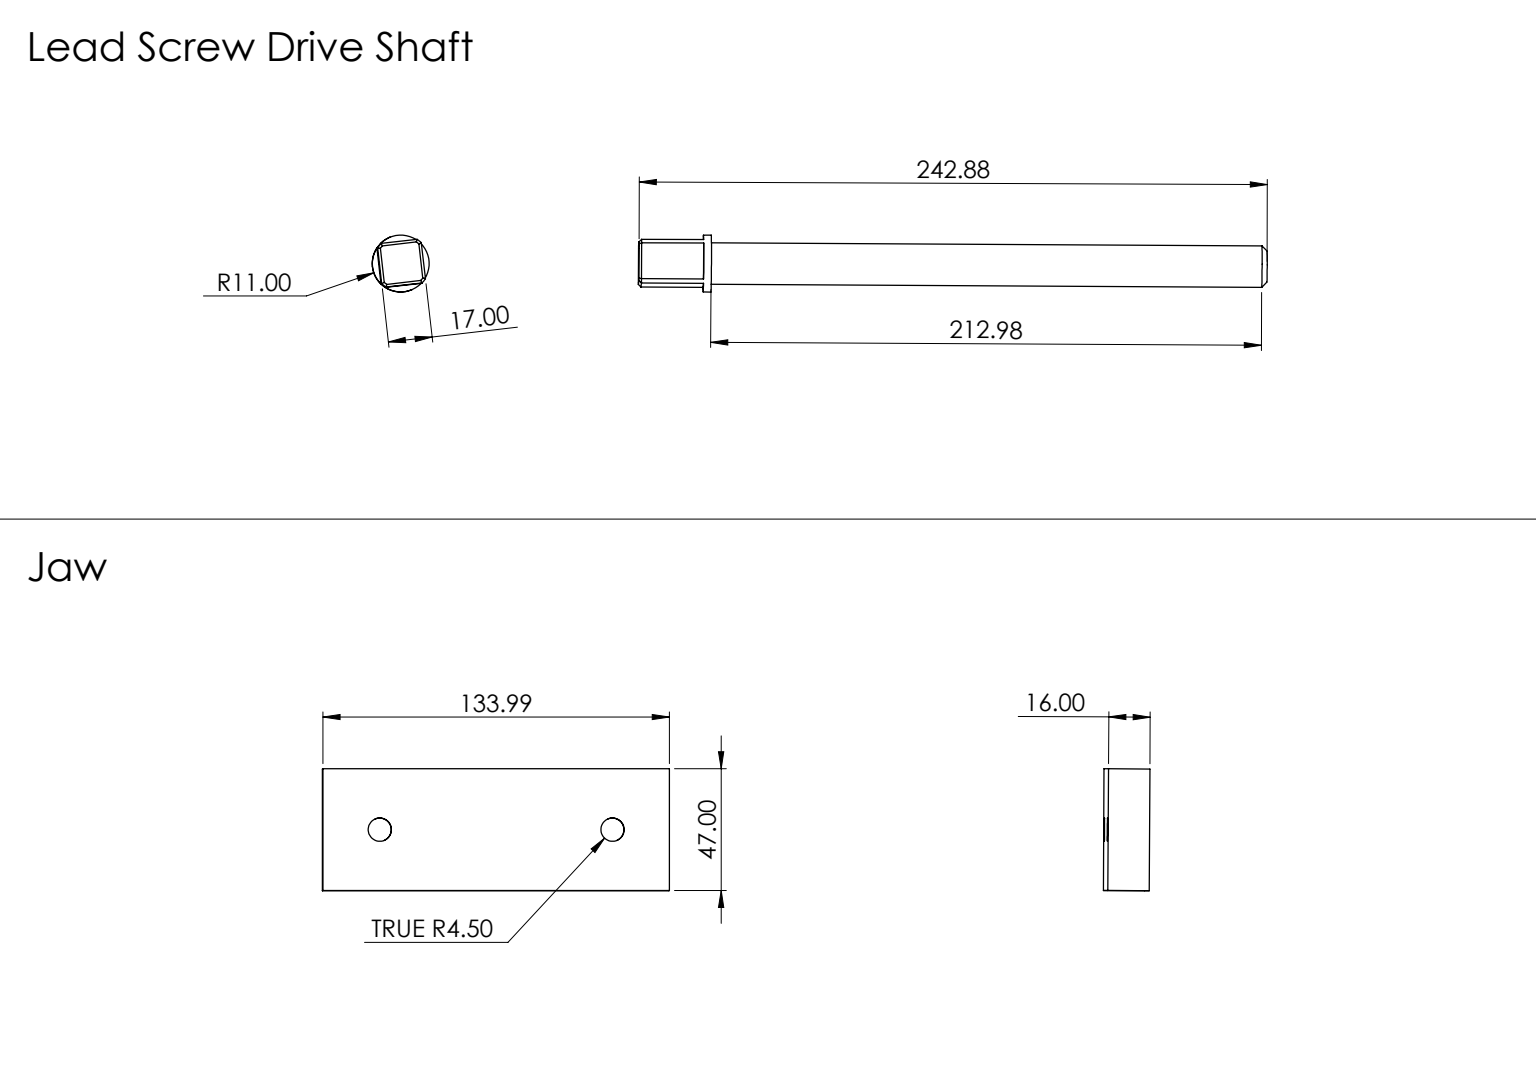
ISO-10303-21;
HEADER;
FILE_DESCRIPTION (('STEP AP214'),
    '1' );
FILE_NAME ('Jaw.step',
    '2026-10-09T10:51:02',
    ( '' ),
    ( '' ),
    'SwSTEP 2.0',
    'SolidWorks 2026',
    '' );
FILE_SCHEMA (( 'AUTOMOTIVE_DESIGN' ));
ENDSEC;

DATA;
#34=DIRECTION ( 'NONE',  ( -7.125109674081160920E-05, 0.9999848031710253382, -0.005512562950849312846 ) ) ;
#150=DIRECTION ( 'NONE',  ( -7.125109674118361251E-05, 0.9999848031710253382, -0.005512562950849477644 ) ) ;
#162=FACE_BOUND ( 'NONE', #20297, .T. ) ;
#274=ORIENTED_EDGE ( 'NONE', *, *, #11916, .F. ) ;
#303=VECTOR ( 'NONE', #7071, 999.9999999999998863 ) ;
#315=CARTESIAN_POINT ( 'NONE',  ( 67.23655452815148692, 145.1029152106949027, 17.86880078497820179 ) ) ;
#352=EDGE_LOOP ( 'NONE', ( #16374, #6015 ) ) ;
#357=ORIENTED_EDGE ( 'NONE', *, *, #20567, .F. ) ;
#370=AXIS2_PLACEMENT_3D ( 'NONE', #9762, #6313, #11942 ) ;
#420=DIRECTION ( 'NONE',  ( -7.125109674025824596E-05, 0.9999848031710253382, -0.005512562950848693549 ) ) ;
#429=LINE ( 'NONE', #2033, #16330 ) ;
#449=AXIS2_PLACEMENT_3D ( 'NONE', #14945, #15170, #16666 ) ;
#652=ORIENTED_EDGE ( 'NONE', *, *, #21301, .F. ) ;
#687=LINE ( 'NONE', #9519, #12271 ) ;
#716=DIRECTION ( 'NONE',  ( -7.125109674025824596E-05, 0.9999848031710253382, -0.005512562950848693549 ) ) ;
#813=UNCERTAINTY_MEASURE_WITH_UNIT (LENGTH_MEASURE( 1.000000000000000082E-05 ), #17647, 'distance_accuracy_value', 'NONE');
#839=VECTOR ( 'NONE', #4920, 999.9999999999998863 ) ;
#857=ORIENTED_EDGE ( 'NONE', *, *, #10212, .F. ) ;
#859=AXIS2_PLACEMENT_3D ( 'NONE', #22163, #3207, #9893 ) ;
#896=DIRECTION ( 'NONE',  ( -7.125109674081160920E-05, 0.9999848031710253382, -0.005512562950849312846 ) ) ;
#960=ADVANCED_FACE ( 'NONE', ( #15043 ), #20731, .F. ) ;
#993=ORIENTED_EDGE ( 'NONE', *, *, #20376, .T. ) ;
#1015=ORIENTED_EDGE ( 'NONE', *, *, #13140, .F. ) ;
#1210=EDGE_CURVE ( 'NONE', #16785, #22481, #5763, .T. ) ;
#1305=CARTESIAN_POINT ( 'NONE',  ( -44.65183966190961939, 161.1467762486291520, 27.22731394492822687 ) ) ;
#1395=DIRECTION ( 'NONE',  ( 1.000000000000000000, 0.000000000000000000, 0.000000000000000000 ) ) ;
#1432=EDGE_LOOP ( 'NONE', ( #10019, #11509, #17070, #14854 ) ) ;
#1475=CARTESIAN_POINT ( 'NONE',  ( 49.83973329503886873, 168.6466622724117599, 25.96463831280822632 ) ) ;
#1540=( GEOMETRIC_REPRESENTATION_CONTEXT ( 3 ) GLOBAL_UNCERTAINTY_ASSIGNED_CONTEXT ( ( #813 ) ) GLOBAL_UNIT_ASSIGNED_CONTEXT ( ( #17647, #10405, #3847 ) ) REPRESENTATION_CONTEXT ( 'NONE', 'WORKASPACE' ) );
#1577=CARTESIAN_POINT ( 'NONE',  ( 45.44318007003697346, 173.1906980738791617, 33.99720069194405170 ) ) ;
#1592=AXIS2_PLACEMENT_3D ( 'NONE', #10762, #9016, #16064 ) ;
#1663=ORIENTED_EDGE ( 'NONE', *, *, #8994, .T. ) ;
#1682=SHAPE_REPRESENTATION_RELATIONSHIP ( 'NONE' , 'NONE' ,  #3137, #19759 ) ;
#1704=LINE ( 'NONE', #11119, #17313 ) ;
#1846=DIRECTION ( 'NONE',  ( -0.01292394549866741384, -0.005513023399720269613, -0.9999012842304692006 ) ) ;
#1876=EDGE_CURVE ( 'NONE', #11555, #17908, #8775, .T. ) ;
#1910=EDGE_CURVE ( 'NONE', #1979, #4369, #21194, .T. ) ;
#1979=VERTEX_POINT ( 'NONE', #8220 ) ;
#1998=PLANE ( 'NONE',  #3714 ) ;
#2033=CARTESIAN_POINT ( 'NONE',  ( 45.23703820192896075, 164.1026264709443865, 18.04839321081418291 ) ) ;
#2042=DIRECTION ( 'NONE',  ( -0.01292394549866741384, -0.005513023399720269613, -0.9999012842304692006 ) ) ;
#2146=CARTESIAN_POINT ( 'NONE',  ( 45.23671757199362986, 168.6025580852140138, 18.02358667753535926 ) ) ;
#2182=ORIENTED_EDGE ( 'NONE', *, *, #8536, .T. ) ;
#2189=CARTESIAN_POINT ( 'NONE',  ( 45.34010913598296355, 168.6466622724117599, 26.02279695137911020 ) ) ;
#2195=CARTESIAN_POINT ( 'NONE',  ( -44.54930311108117280, 173.1906980738792186, 35.16037346336178615 ) ) ;
#2208=ORIENTED_EDGE ( 'NONE', *, *, #19527, .F. ) ;
#2265=AXIS2_PLACEMENT_3D ( 'NONE', #6781, #4820, #15212 ) ;
#2299=AXIS2_PLACEMENT_3D ( 'NONE', #18895, #10594, #12683 ) ;
#2309=VERTEX_POINT ( 'NONE', #20349 ) ;
#2386=CARTESIAN_POINT ( 'NONE',  ( 0.4472591094132349898, 168.6907664596095628, 34.60359361093173902 ) ) ;
#2477=CARTESIAN_POINT ( 'NONE',  ( -66.75225376373553843, 145.1029152106950164, 19.60063580020017326 ) ) ;
#2488=DIRECTION ( 'NONE',  ( -0.01292394549866741384, -0.005513023399720270480, -0.9999012842304693116 ) ) ;
#2502=DIRECTION ( 'NONE',  ( 0.01292394549866741557, 0.005513023399720270480, 0.9999012842304693116 ) ) ;
#2503=EDGE_CURVE ( 'NONE', #1979, #11555, #13540, .T. ) ;
#2515=DIRECTION ( 'NONE',  ( -7.125109674025824596E-05, 0.9999848031710253382, -0.005512562950849464634 ) ) ;
#2611=ADVANCED_FACE ( 'NONE', ( #19733 ), #11028, .F. ) ;
#2640=DIRECTION ( 'NONE',  ( -7.125109674118361251E-05, 0.9999848031710253382, -0.005512562950849477644 ) ) ;
#2688=EDGE_CURVE ( 'NONE', #17908, #4369, #17967, .T. ) ;
#2724=FACE_OUTER_BOUND ( 'NONE', #16793, .T. ) ;
#2742=EDGE_LOOP ( 'NONE', ( #5687, #11839, #12737, #13981 ) ) ;
#2858=DIRECTION ( 'NONE',  ( -0.01292394549866741384, -0.005513023399720269613, -0.9999012842304692006 ) ) ;
#2946=CARTESIAN_POINT ( 'NONE',  ( -44.75576560912451640, 168.6025580852140706, 19.18675944895310082 ) ) ;
#2950=AXIS2_PLACEMENT_3D ( 'NONE', #15940, #17886, #10862 ) ;
#2958=DIRECTION ( 'NONE',  ( 7.125109674081160920E-05, -0.9999848031710253382, 0.005512562950849312846 ) ) ;
#3047=CARTESIAN_POINT ( 'NONE',  ( -44.75576560912451640, 168.6025580852140706, 19.18675944895310082 ) ) ;
#3102=CARTESIAN_POINT ( 'NONE',  ( 0.000000000000000000, 0.000000000000000000, 0.000000000000000000 ) ) ;
#3137=SHAPE_REPRESENTATION ( 'Jaw', ( #6292 ), #1540 ) ;
#3142=ORIENTED_EDGE ( 'NONE', *, *, #1210, .T. ) ;
#3161=DIRECTION ( 'NONE',  ( 0.9999164797902015955, -8.863511990578706951E-16, -0.01292414190464158050 ) ) ;
#3206=ORIENTED_EDGE ( 'NONE', *, *, #18469, .T. ) ;
#3207=DIRECTION ( 'NONE',  ( 0.9999164797902017066, -7.828075210616901716E-16, -0.01292414190464158050 ) ) ;
#3223=FILL_AREA_STYLE_COLOUR ( '', #5839 ) ;
#3229=ADVANCED_FACE ( 'NONE', ( #17210 ), #13216, .F. ) ;
#3262=CLOSED_SHELL ( 'NONE', ( #960, #13040, #16685, #12758, #12715, #2611, #14277, #3229, #16518, #17138, #11889, #12219, #12513, #10902, #16471, #20249 ) ) ;
#3290=CARTESIAN_POINT ( 'NONE',  ( -66.54881943730367766, 192.1904093341287307, 35.33996588919776372 ) ) ;
#3509=ORIENTED_EDGE ( 'NONE', *, *, #8994, .F. ) ;
#3589=PLANE ( 'NONE',  #6302 ) ;
#3714=AXIS2_PLACEMENT_3D ( 'NONE', #7158, #7374, #14069 ) ;
#3790=ORIENTED_EDGE ( 'NONE', *, *, #16760, .F. ) ;
#3796=DIRECTION ( 'NONE',  ( 7.125109674070808144E-05, -0.9999848031710253382, 0.005512562950849314580 ) ) ;
#3829=ORIENTED_EDGE ( 'NONE', *, *, #21301, .T. ) ;
#3831=APPLICATION_CONTEXT ( 'automotive_design' ) ;
#3847=( NAMED_UNIT ( * ) SI_UNIT ( $, .STERADIAN. ) SOLID_ANGLE_UNIT ( ) );
#3860=DIRECTION ( 'NONE',  ( -0.01292394549866741384, -0.005513023399720269613, -0.9999012842304692006 ) ) ;
#3866=CARTESIAN_POINT ( 'NONE',  ( 67.43998885458336190, 192.1904093341285886, 33.60813087397579579 ) ) ;
#3913=ORIENTED_EDGE ( 'NONE', *, *, #21314, .T. ) ;
#3924=FACE_BOUND ( 'NONE', #15682, .T. ) ;
#3930=EDGE_CURVE ( 'NONE', #2309, #13637, #6615, .T. ) ;
#4026=CARTESIAN_POINT ( 'NONE',  ( 45.34010913598296355, 168.6466622724117599, 26.02279695137911020 ) ) ;
#4040=VECTOR ( 'NONE', #34, 999.9999999999998863 ) ;
#4114=ORIENTED_EDGE ( 'NONE', *, *, #11916, .T. ) ;
#4250=DIRECTION ( 'NONE',  ( -0.01292394549866741384, -0.005513023399720269613, -0.9999012842304692006 ) ) ;
#4369=VERTEX_POINT ( 'NONE', #10030 ) ;
#4422=FACE_BOUND ( 'NONE', #352, .T. ) ;
#4509=DIRECTION ( 'NONE',  ( -0.9999164797902015955, 8.863511990578706951E-16, 0.01292414190464158050 ) ) ;
#4565=CARTESIAN_POINT ( 'NONE',  ( 67.43998885458336190, 192.1904093341285886, 33.60813087397579579 ) ) ;
#4603=DIRECTION ( 'NONE',  ( -0.01292394549866741384, -0.005513023399720269613, -0.9999012842304692006 ) ) ;
#4820=DIRECTION ( 'NONE',  ( -0.01292394549866741384, -0.005513023399720269613, -0.9999012842304692006 ) ) ;
#4851=CARTESIAN_POINT ( 'NONE',  ( -66.75225376373553843, 145.1029152106950164, 19.60063580020017326 ) ) ;
#4882=CARTESIAN_POINT ( 'NONE',  ( 67.23320572660466610, 192.1022009597330680, 17.60971032628828681 ) ) ;
#4920=DIRECTION ( 'NONE',  ( 0.01292394549866741557, 0.005513023399720270480, 0.9999012842304693116 ) ) ;
#4939=DIRECTION ( 'NONE',  ( -7.125109674025824596E-05, 0.9999848031710253382, -0.005512562950848693549 ) ) ;
#5024=LINE ( 'NONE', #19276, #839 ) ;
#5123=DIRECTION ( 'NONE',  ( -0.01292394549866741557, -0.005513023399720270480, -0.9999012842304693116 ) ) ;
#5172=CARTESIAN_POINT ( 'NONE',  ( 45.33978850604763977, 173.1465938866814156, 25.99799041810029010 ) ) ;
#5189=DIRECTION ( 'NONE',  ( -7.125109674118361251E-05, 0.9999848031710253382, -0.005512562950849477644 ) ) ;
#5192=FACE_OUTER_BOUND ( 'NONE', #8383, .T. ) ;
#5241=VECTOR ( 'NONE', #9729, 999.9999999999998863 ) ;
#5244=CARTESIAN_POINT ( 'NONE',  ( 67.23320572660466610, 192.1022009597330680, 17.60971032628828681 ) ) ;
#5302=ORIENTED_EDGE ( 'NONE', *, *, #18906, .T. ) ;
#5343=EDGE_LOOP ( 'NONE', ( #12524, #5537, #17319, #2208 ) ) ;
#5409=CARTESIAN_POINT ( 'NONE',  ( -66.75560256528235925, 192.1022009597331817, 19.34154534151025118 ) ) ;
#5448=CARTESIAN_POINT ( 'NONE',  ( -44.75544497918918552, 164.1026264709444433, 19.21156598223192447 ) ) ;
#5473=( GEOMETRIC_REPRESENTATION_CONTEXT ( 3 ) GLOBAL_UNCERTAINTY_ASSIGNED_CONTEXT ( ( #16447 ) ) GLOBAL_UNIT_ASSIGNED_CONTEXT ( ( #13592, #10248, #6903 ) ) REPRESENTATION_CONTEXT ( 'NONE', 'WORKASPACE' ) );
#5530=DIRECTION ( 'NONE',  ( -0.01292394549866741384, -0.005513023399720269613, -0.9999012842304692006 ) ) ;
#5536=DIRECTION ( 'NONE',  ( -7.125109674081160920E-05, 0.9999848031710253382, -0.005512562950849312846 ) ) ;
#5537=ORIENTED_EDGE ( 'NONE', *, *, #15039, .T. ) ;
#5601=DIRECTION ( 'NONE',  ( -0.01292394549866741557, -0.005513023399720270480, -0.9999012842304693116 ) ) ;
#5633=ORIENTED_EDGE ( 'NONE', *, *, #8536, .F. ) ;
#5687=ORIENTED_EDGE ( 'NONE', *, *, #21314, .F. ) ;
#5699=ORIENTED_EDGE ( 'NONE', *, *, #8354, .T. ) ;
#5710=CARTESIAN_POINT ( 'NONE',  ( 45.23725195521918607, 161.1026720614313206, 18.06493089966673082 ) ) ;
#5763=CIRCLE ( 'NONE', #9429, 7.499999999999992006 ) ;
#5779=ORIENTED_EDGE ( 'NONE', *, *, #5841, .F. ) ;
#5799=CARTESIAN_POINT ( 'NONE',  ( -44.65237404513518271, 168.6466622724118452, 27.18596972279685531 ) ) ;
#5839=COLOUR_RGB ( '', 0.66274510, 0.83137255, 0.94901961) ;
#5841=EDGE_CURVE ( 'NONE', #22481, #16785, #12846, .T. ) ;
#5869=DIRECTION ( 'NONE',  ( 0.01292394549866741557, 0.005513023399720270480, 0.9999012842304693116 ) ) ;
#5948=VERTEX_POINT ( 'NONE', #3866 ) ;
#6015=ORIENTED_EDGE ( 'NONE', *, *, #2503, .T. ) ;
#6040=DIRECTION ( 'NONE',  ( 0.01292394549866741557, 0.005513023399720270480, 0.9999012842304693116 ) ) ;
#6066=EDGE_LOOP ( 'NONE', ( #17206, #11430, #22627, #3829 ) ) ;
#6141=VERTEX_POINT ( 'NONE', #19233 ) ;
#6248=PRODUCT_DEFINITION_SHAPE ( 'NONE', 'NONE',  #18701 ) ;
#6262=EDGE_LOOP ( 'NONE', ( #19835, #11435, #16456, #17358 ) ) ;
#6292=AXIS2_PLACEMENT_3D ( 'NONE', #3102, #12069, #1395 ) ;
#6302=AXIS2_PLACEMENT_3D ( 'NONE', #12228, #14296, #5536 ) ;
#6313=DIRECTION ( 'NONE',  ( -7.125109674070808144E-05, 0.9999848031710253382, -0.005512562950849314580 ) ) ;
#6355=VECTOR ( 'NONE', #6651, 999.9999999999998863 ) ;
#6463=VECTOR ( 'NONE', #15305, 1000.000000000000227 ) ;
#6479=CARTESIAN_POINT ( 'NONE',  ( 67.23655452815148692, 145.1029152106949027, 17.86880078497820179 ) ) ;
#6524=ORIENTED_EDGE ( 'NONE', *, *, #10212, .T. ) ;
#6562=CYLINDRICAL_SURFACE ( 'NONE', #2265, 7.499999999999992006 ) ;
#6613=EDGE_CURVE ( 'NONE', #20796, #7407, #16201, .T. ) ;
#6615=LINE ( 'NONE', #4882, #13876 ) ;
#6616=ORIENTED_EDGE ( 'NONE', *, *, #2503, .F. ) ;
#6651=DIRECTION ( 'NONE',  ( -0.01292394549866741557, -0.005513023399720270480, -0.9999012842304693116 ) ) ;
#6654=DIRECTION ( 'NONE',  ( -7.125109674118361251E-05, 0.9999848031710253382, -0.005512562950849477644 ) ) ;
#6699=VERTEX_POINT ( 'NONE', #15288 ) ;
#6700=CIRCLE ( 'NONE', #19532, 7.499999999999992006 ) ;
#6781=CARTESIAN_POINT ( 'NONE',  ( 45.23671757199362986, 168.6025580852140138, 18.02358667753535926 ) ) ;
#6824=EDGE_CURVE ( 'NONE', #11456, #16120, #12038, .T. ) ;
#6889=EDGE_CURVE ( 'NONE', #16785, #10445, #1704, .T. ) ;
#6903=( NAMED_UNIT ( * ) SI_UNIT ( $, .STERADIAN. ) SOLID_ANGLE_UNIT ( ) );
#6983=CIRCLE ( 'NONE', #2950, 4.500000000000006217 ) ;
#6989=AXIS2_PLACEMENT_3D ( 'NONE', #4026, #16369, #21485 ) ;
#7027=ORIENTED_EDGE ( 'NONE', *, *, #6889, .F. ) ;
#7071=DIRECTION ( 'NONE',  ( -0.01292394549866741557, -0.005513023399720270480, -0.9999012842304693116 ) ) ;
#7104=CARTESIAN_POINT ( 'NONE',  ( 45.44382132990763523, 164.1908348453399071, 34.04681375850169189 ) ) ;
#7156=LINE ( 'NONE', #5409, #4040 ) ;
#7158=CARTESIAN_POINT ( 'NONE',  ( -40.15274988607927042, 168.6466622724118452, 27.12781108422596787 ) ) ;
#7369=FACE_OUTER_BOUND ( 'NONE', #15788, .T. ) ;
#7374=DIRECTION ( 'NONE',  ( 0.01292394549866741384, 0.005513023399720270480, 0.9999012842304693116 ) ) ;
#7407=VERTEX_POINT ( 'NONE', #5172 ) ;
#7545=DIRECTION ( 'NONE',  ( -0.01292394549866741557, -0.005513023399720270480, -0.9999012842304693116 ) ) ;
#7554=DIRECTION ( 'NONE',  ( -7.125109674118361251E-05, 0.9999848031710253382, -0.005512562950849477644 ) ) ;
#7597=CARTESIAN_POINT ( 'NONE',  ( -66.75560256528235925, 192.1022009597331817, 19.34154534151025118 ) ) ;
#7693=EDGE_LOOP ( 'NONE', ( #1663, #3913 ) ) ;
#7826=CIRCLE ( 'NONE', #20652, 4.500000000000006217 ) ;
#7827=CARTESIAN_POINT ( 'NONE',  ( -44.75576560912451640, 168.6025580852140706, 19.18675944895310082 ) ) ;
#7956=EDGE_CURVE ( 'NONE', #8451, #10445, #6700, .T. ) ;
#8109=DIRECTION ( 'NONE',  ( -7.125109674025824596E-05, 0.9999848031710253382, -0.005512562950849464634 ) ) ;
#8121=ORIENTED_EDGE ( 'NONE', *, *, #19527, .T. ) ;
#8134=VECTOR ( 'NONE', #2958, 999.9999999999998863 ) ;
#8201=LINE ( 'NONE', #6479, #21757 ) ;
#8220=CARTESIAN_POINT ( 'NONE',  ( -44.54866185121051103, 164.1908348453399640, 35.20998652991943345 ) ) ;
#8272=LINE ( 'NONE', #14961, #6463 ) ;
#8274=ORIENTED_EDGE ( 'NONE', *, *, #1910, .F. ) ;
#8354=EDGE_CURVE ( 'NONE', #22481, #8451, #15395, .T. ) ;
#8359=PRODUCT_CONTEXT ( 'NONE', #16460, 'mechanical' ) ;
#8363=CARTESIAN_POINT ( 'NONE',  ( 45.23639694205829898, 173.1024896994836411, 17.99878014425653561 ) ) ;
#8383=EDGE_LOOP ( 'NONE', ( #9522, #15270, #4114, #12068 ) ) ;
#8385=FACE_OUTER_BOUND ( 'NONE', #5343, .T. ) ;
#8451=VERTEX_POINT ( 'NONE', #17687 ) ;
#8454=PLANE ( 'NONE',  #19947 ) ;
#8456=DIRECTION ( 'NONE',  ( -7.125109674081160920E-05, 0.9999848031710253382, -0.005512562950849312846 ) ) ;
#8511=SURFACE_SIDE_STYLE ('',( #13710 ) ) ;
#8536=EDGE_CURVE ( 'NONE', #6699, #8927, #9159, .T. ) ;
#8600=ORIENTED_EDGE ( 'NONE', *, *, #19467, .T. ) ;
#8609=EDGE_LOOP ( 'NONE', ( #6616, #18782, #8600, #15706 ) ) ;
#8637=FACE_OUTER_BOUND ( 'NONE', #14758, .T. ) ;
#8656=EDGE_CURVE ( 'NONE', #16120, #5948, #9743, .T. ) ;
#8676=CARTESIAN_POINT ( 'NONE',  ( 67.44333765613016851, 145.1911235850904234, 33.86722133266570722 ) ) ;
#8696=DIRECTION ( 'NONE',  ( -0.01292394549866741384, -0.005513023399720269613, -0.9999012842304692006 ) ) ;
#8763=STYLED_ITEM ( 'NONE', ( #22281 ), #17335 ) ;
#8775=LINE ( 'NONE', #12378, #303 ) ;
#8802=EDGE_LOOP ( 'NONE', ( #12427, #652, #17135, #3206 ) ) ;
#8858=DIRECTION ( 'NONE',  ( -0.01292394549866741384, -0.005513023399720269613, -0.9999012842304692006 ) ) ;
#8909=ORIENTED_EDGE ( 'NONE', *, *, #20376, .F. ) ;
#8927=VERTEX_POINT ( 'NONE', #21509 ) ;
#8975=CARTESIAN_POINT ( 'NONE',  ( -44.65237404513518271, 168.6466622724118452, 27.18596972279685531 ) ) ;
#8994=EDGE_CURVE ( 'NONE', #12945, #18985, #6983, .T. ) ;
#9016=DIRECTION ( 'NONE',  ( -0.01292394549866741384, -0.005513023399720269613, -0.9999012842304692006 ) ) ;
#9046=DIRECTION ( 'NONE',  ( -0.01292394549866741384, -0.005513023399720269613, -0.9999012842304692006 ) ) ;
#9159=CIRCLE ( 'NONE', #14347, 7.499999999999992006 ) ;
#9239=VECTOR ( 'NONE', #6040, 999.9999999999998863 ) ;
#9339=VERTEX_POINT ( 'NONE', #315 ) ;
#9429=AXIS2_PLACEMENT_3D ( 'NONE', #8975, #8858, #150 ) ;
#9442=ORIENTED_EDGE ( 'NONE', *, *, #18345, .F. ) ;
#9494=CARTESIAN_POINT ( 'NONE',  ( 67.43998885458336190, 192.1904093341285886, 33.60813087397579579 ) ) ;
#9519=CARTESIAN_POINT ( 'NONE',  ( 67.23320572660466610, 192.1022009597330680, 17.60971032628828681 ) ) ;
#9522=ORIENTED_EDGE ( 'NONE', *, *, #15583, .T. ) ;
#9603=LINE ( 'NONE', #2477, #9239 ) ;
#9676=DIRECTION ( 'NONE',  ( -0.01292394549866741384, -0.005513023399720269613, -0.9999012842304692006 ) ) ;
#9682=AXIS2_PLACEMENT_3D ( 'NONE', #3047, #10069, #8109 ) ;
#9683=ORIENTED_EDGE ( 'NONE', *, *, #15039, .F. ) ;
#9729=DIRECTION ( 'NONE',  ( -0.01292394549866741557, -0.005513023399720270480, -0.9999012842304693116 ) ) ;
#9743=LINE ( 'NONE', #9494, #20554 ) ;
#9762=CARTESIAN_POINT ( 'NONE',  ( 67.23655452815148692, 145.1029152106949027, 17.86880078497820179 ) ) ;
#9768=SHAPE_DEFINITION_REPRESENTATION ( #6248, #3137 ) ;
#9893=DIRECTION ( 'NONE',  ( 7.125109674081160920E-05, -0.9999848031710253382, 0.005512562950849312846 ) ) ;
#10013=CARTESIAN_POINT ( 'NONE',  ( 45.23671757199362986, 168.6025580852140138, 18.02358667753535926 ) ) ;
#10019=ORIENTED_EDGE ( 'NONE', *, *, #1210, .F. ) ;
#10030=CARTESIAN_POINT ( 'NONE',  ( -44.65205341519984472, 164.1467306581422179, 27.21077625607567541 ) ) ;
#10069=DIRECTION ( 'NONE',  ( -0.01292394549866741384, -0.005513023399720269613, -0.9999012842304692006 ) ) ;
#10076=ORIENTED_EDGE ( 'NONE', *, *, #19467, .F. ) ;
#10186=PRODUCT_DEFINITION_CONTEXT ( 'detailed design', #3831, 'design' ) ;
#10204=CARTESIAN_POINT ( 'NONE',  ( -44.75629999235007972, 176.1024441089967638, 19.14541522682172925 ) ) ;
#10212=EDGE_CURVE ( 'NONE', #6141, #15758, #14916, .T. ) ;
#10234=DIRECTION ( 'NONE',  ( -7.125109674025824596E-05, 0.9999848031710253382, -0.005512562950849464634 ) ) ;
#10248=( NAMED_UNIT ( * ) PLANE_ANGLE_UNIT ( ) SI_UNIT ( $, .RADIAN. ) );
#10320=CARTESIAN_POINT ( 'NONE',  ( 45.34064351920852687, 161.1467762486290951, 26.06414117351048176 ) ) ;
#10405=( NAMED_UNIT ( * ) PLANE_ANGLE_UNIT ( ) SI_UNIT ( $, .RADIAN. ) );
#10445=VERTEX_POINT ( 'NONE', #18712 ) ;
#10482=SURFACE_STYLE_USAGE ( .BOTH. , #8511 ) ;
#10529=EDGE_CURVE ( 'NONE', #12252, #11456, #8272, .T. ) ;
#10594=DIRECTION ( 'NONE',  ( -0.01292394549866741384, -0.005513023399720269613, -0.9999012842304692006 ) ) ;
#10610=AXIS2_PLACEMENT_3D ( 'NONE', #19850, #3796, #17840 ) ;
#10643=DIRECTION ( 'NONE',  ( -7.125109674118361251E-05, 0.9999848031710253382, -0.005512562950849477644 ) ) ;
#10730=VECTOR ( 'NONE', #5601, 999.9999999999998863 ) ;
#10762=CARTESIAN_POINT ( 'NONE',  ( -44.65237404513518271, 168.6466622724118452, 27.18596972279685531 ) ) ;
#10832=CARTESIAN_POINT ( 'NONE',  ( -44.65290842836073182, 176.1465482961945384, 27.14462550066548729 ) ) ;
#10862=DIRECTION ( 'NONE',  ( -7.125109674025824596E-05, 0.9999848031710253382, -0.005512562950848693549 ) ) ;
#10902=ADVANCED_FACE ( 'NONE', ( #18665 ), #20491, .F. ) ;
#10944=ORIENTED_EDGE ( 'NONE', *, *, #7956, .T. ) ;
#10995=ORIENTED_EDGE ( 'NONE', *, *, #2688, .T. ) ;
#11005=VECTOR ( 'NONE', #5123, 999.9999999999998863 ) ;
#11028=PLANE ( 'NONE',  #10610 ) ;
#11094=VECTOR ( 'NONE', #2502, 999.9999999999998863 ) ;
#11114=FACE_BOUND ( 'NONE', #7693, .T. ) ;
#11119=CARTESIAN_POINT ( 'NONE',  ( -44.75523122589896019, 161.1026720614313774, 19.22810367108447238 ) ) ;
#11145=ORIENTED_EDGE ( 'NONE', *, *, #18345, .T. ) ;
#11216=EDGE_CURVE ( 'NONE', #9339, #16395, #8201, .T. ) ;
#11345=LINE ( 'NONE', #12849, #11094 ) ;
#11362=DIRECTION ( 'NONE',  ( -0.01292394549866741384, -0.005513023399720269613, -0.9999012842304692006 ) ) ;
#11381=DIRECTION ( 'NONE',  ( -0.01292394549866741384, -0.005513023399720269613, -0.9999012842304692006 ) ) ;
#11430=ORIENTED_EDGE ( 'NONE', *, *, #18879, .F. ) ;
#11435=ORIENTED_EDGE ( 'NONE', *, *, #18469, .F. ) ;
#11442=ORIENTED_EDGE ( 'NONE', *, *, #15094, .F. ) ;
#11456=VERTEX_POINT ( 'NONE', #20925 ) ;
#11486=CARTESIAN_POINT ( 'NONE',  ( 45.34010913598296355, 168.6466622724117599, 26.02279695137911020 ) ) ;
#11509=ORIENTED_EDGE ( 'NONE', *, *, #6889, .T. ) ;
#11555=VERTEX_POINT ( 'NONE', #2195 ) ;
#11630=DIRECTION ( 'NONE',  ( -7.125109674118361251E-05, 0.9999848031710253382, -0.005512562950849477644 ) ) ;
#11689=CYLINDRICAL_SURFACE ( 'NONE', #15178, 4.500000000000006217 ) ;
#11839=ORIENTED_EDGE ( 'NONE', *, *, #20567, .T. ) ;
#11856=PLANE ( 'NONE',  #859 ) ;
#11889=ADVANCED_FACE ( 'NONE', ( #19839 ), #14832, .F. ) ;
#11916=EDGE_CURVE ( 'NONE', #13637, #9339, #687, .T. ) ;
#11942=DIRECTION ( 'NONE',  ( 0.9999164797902015955, -8.863511990578707937E-16, -0.01292414190464158050 ) ) ;
#12038=LINE ( 'NONE', #3290, #12545 ) ;
#12068=ORIENTED_EDGE ( 'NONE', *, *, #11216, .T. ) ;
#12069=DIRECTION ( 'NONE',  ( 0.000000000000000000, 0.000000000000000000, 1.000000000000000000 ) ) ;
#12199=CIRCLE ( 'NONE', #449, 7.499999999999992006 ) ;
#12219=ADVANCED_FACE ( 'NONE', ( #17448, #21095 ), #8454, .F. ) ;
#12228=CARTESIAN_POINT ( 'NONE',  ( 0.2404759814345563407, 168.6025580852140422, 18.60517306324423004 ) ) ;
#12252=VERTEX_POINT ( 'NONE', #8676 ) ;
#12271=VECTOR ( 'NONE', #19960, 999.9999999999998863 ) ;
#12289=DIRECTION ( 'NONE',  ( -0.9999164797902017066, 7.828075210616901716E-16, 0.01292414190464158050 ) ) ;
#12302=ORIENTED_EDGE ( 'NONE', *, *, #15632, .T. ) ;
#12378=CARTESIAN_POINT ( 'NONE',  ( -44.75608623905984729, 173.1024896994836979, 19.16195291567427716 ) ) ;
#12427=ORIENTED_EDGE ( 'NONE', *, *, #6824, .T. ) ;
#12451=FACE_BOUND ( 'NONE', #20432, .T. ) ;
#12484=DIRECTION ( 'NONE',  ( -0.01292394549866741557, -0.005513023399720270480, -0.9999012842304693116 ) ) ;
#12513=ADVANCED_FACE ( 'NONE', ( #7369 ), #19321, .F. ) ;
#12524=ORIENTED_EDGE ( 'NONE', *, *, #15632, .F. ) ;
#12545=VECTOR ( 'NONE', #8456, 999.9999999999998863 ) ;
#12683=DIRECTION ( 'NONE',  ( -7.125109674118361251E-05, 0.9999848031710253382, -0.005512562950849477644 ) ) ;
#12715=ADVANCED_FACE ( 'NONE', ( #18618 ), #11856, .F. ) ;
#12737=ORIENTED_EDGE ( 'NONE', *, *, #6613, .T. ) ;
#12758=ADVANCED_FACE ( 'NONE', ( #22264 ), #15424, .F. ) ;
#12846=CIRCLE ( 'NONE', #21246, 7.499999999999992006 ) ;
#12849=CARTESIAN_POINT ( 'NONE',  ( 67.23655452815148692, 145.1029152106949027, 17.86880078497820179 ) ) ;
#12945=VERTEX_POINT ( 'NONE', #1577 ) ;
#13021=DIRECTION ( 'NONE',  ( -7.125109674118361251E-05, 0.9999848031710253382, -0.005512562950849477644 ) ) ;
#13040=ADVANCED_FACE ( 'NONE', ( #13428 ), #11689, .F. ) ;
#13140=EDGE_CURVE ( 'NONE', #11555, #1979, #7826, .T. ) ;
#13216=PLANE ( 'NONE',  #370 ) ;
#13242=PRODUCT_DEFINITION_FORMATION_WITH_SPECIFIED_SOURCE ( 'ANY', '', #18549, .NOT_KNOWN. ) ;
#13244=CARTESIAN_POINT ( 'NONE',  ( 45.44350069997230435, 168.6907664596095344, 34.02200722522286469 ) ) ;
#13428=FACE_OUTER_BOUND ( 'NONE', #8609, .T. ) ;
#13540=CIRCLE ( 'NONE', #19391, 4.500000000000006217 ) ;
#13592=( LENGTH_UNIT ( ) NAMED_UNIT ( * ) SI_UNIT ( .MILLI., .METRE. ) );
#13637=VERTEX_POINT ( 'NONE', #14988 ) ;
#13710=SURFACE_STYLE_FILL_AREA ( #22607 ) ;
#13846=DIRECTION ( 'NONE',  ( -7.125109674118361251E-05, 0.9999848031710253382, -0.005512562950849477644 ) ) ;
#13876=VECTOR ( 'NONE', #3161, 1000.000000000000227 ) ;
#13939=CARTESIAN_POINT ( 'NONE',  ( 45.34010913598296355, 168.6466622724117599, 26.02279695137911020 ) ) ;
#13981=ORIENTED_EDGE ( 'NONE', *, *, #18906, .F. ) ;
#13996=ORIENTED_EDGE ( 'NONE', *, *, #16983, .F. ) ;
#14069=DIRECTION ( 'NONE',  ( 7.125109674081160920E-05, -0.9999848031710253382, 0.005512562950849312846 ) ) ;
#14117=CIRCLE ( 'NONE', #17060, 4.500000000000006217 ) ;
#14277=ADVANCED_FACE ( 'NONE', ( #21515 ), #21107, .F. ) ;
#14296=DIRECTION ( 'NONE',  ( -0.01292394549866741384, -0.005513023399720270480, -0.9999012842304693116 ) ) ;
#14347=AXIS2_PLACEMENT_3D ( 'NONE', #2146, #2042, #7554 ) ;
#14413=AXIS2_PLACEMENT_3D ( 'NONE', #16919, #4603, #11630 ) ;
#14485=LINE ( 'NONE', #5710, #10730 ) ;
#14544=AXIS2_PLACEMENT_3D ( 'NONE', #11486, #11362, #2640 ) ;
#14696=ORIENTED_EDGE ( 'NONE', *, *, #18879, .T. ) ;
#14758=EDGE_LOOP ( 'NONE', ( #22103, #3142 ) ) ;
#14832=CYLINDRICAL_SURFACE ( 'NONE', #15591, 4.500000000000006217 ) ;
#14854=ORIENTED_EDGE ( 'NONE', *, *, #8354, .F. ) ;
#14916=CIRCLE ( 'NONE', #14544, 7.499999999999992006 ) ;
#14945=CARTESIAN_POINT ( 'NONE',  ( -44.75576560912451640, 168.6025580852140706, 19.18675944895310082 ) ) ;
#14952=DIRECTION ( 'NONE',  ( -7.125109674025824596E-05, 0.9999848031710253382, -0.005512562950849464634 ) ) ;
#14961=CARTESIAN_POINT ( 'NONE',  ( 67.44333765613016851, 145.1911235850904234, 33.86722133266570722 ) ) ;
#14962=FACE_OUTER_BOUND ( 'NONE', #19645, .T. ) ;
#14988=CARTESIAN_POINT ( 'NONE',  ( 67.23320572660466610, 192.1022009597330680, 17.60971032628828681 ) ) ;
#15039=EDGE_CURVE ( 'NONE', #15758, #8927, #14485, .T. ) ;
#15043=FACE_OUTER_BOUND ( 'NONE', #1432, .T. ) ;
#15055=ORIENTED_EDGE ( 'NONE', *, *, #1876, .T. ) ;
#15094=EDGE_CURVE ( 'NONE', #9339, #12252, #11345, .T. ) ;
#15170=DIRECTION ( 'NONE',  ( -0.01292394549866741384, -0.005513023399720269613, -0.9999012842304692006 ) ) ;
#15178=AXIS2_PLACEMENT_3D ( 'NONE', #2946, #15276, #20510 ) ;
#15192=CIRCLE ( 'NONE', #1592, 4.500000000000006217 ) ;
#15212=DIRECTION ( 'NONE',  ( -7.125109674118361251E-05, 0.9999848031710253382, -0.005512562950849477644 ) ) ;
#15270=ORIENTED_EDGE ( 'NONE', *, *, #3930, .T. ) ;
#15276=DIRECTION ( 'NONE',  ( -0.01292394549866741384, -0.005513023399720269613, -0.9999012842304692006 ) ) ;
#15288=CARTESIAN_POINT ( 'NONE',  ( 45.23618318876806654, 176.1024441089967070, 17.98224245540398769 ) ) ;
#15305=DIRECTION ( 'NONE',  ( -0.9999164797902015955, 8.863511990578706951E-16, 0.01292414190464158050 ) ) ;
#15395=LINE ( 'NONE', #10204, #11005 ) ;
#15424=CYLINDRICAL_SURFACE ( 'NONE', #21385, 4.500000000000006217 ) ;
#15479=DIRECTION ( 'NONE',  ( -0.01292394549866741384, -0.005513023399720269613, -0.9999012842304692006 ) ) ;
#15503=DIRECTION ( 'NONE',  ( 0.01292394549866741384, 0.005513023399720270480, 0.9999012842304693116 ) ) ;
#15511=DIRECTION ( 'NONE',  ( -7.125109674081160920E-05, 0.9999848031710253382, -0.005512562950849312846 ) ) ;
#15583=EDGE_CURVE ( 'NONE', #16395, #2309, #7156, .T. ) ;
#15591=AXIS2_PLACEMENT_3D ( 'NONE', #18160, #9046, #2515 ) ;
#15632=EDGE_CURVE ( 'NONE', #15758, #6141, #19803, .T. ) ;
#15682=EDGE_LOOP ( 'NONE', ( #5633, #3790 ) ) ;
#15699=AXIS2_PLACEMENT_3D ( 'NONE', #18998, #15479, #13846 ) ;
#15706=ORIENTED_EDGE ( 'NONE', *, *, #1876, .F. ) ;
#15747=CARTESIAN_POINT ( 'NONE',  ( -44.75576560912451640, 168.6025580852140706, 19.18675944895310082 ) ) ;
#15758=VERTEX_POINT ( 'NONE', #10320 ) ;
#15762=ORIENTED_EDGE ( 'NONE', *, *, #8656, .F. ) ;
#15788=EDGE_LOOP ( 'NONE', ( #9683, #857, #8121, #2182 ) ) ;
#15814=AXIS2_PLACEMENT_3D ( 'NONE', #13939, #5530, #5189 ) ;
#15940=CARTESIAN_POINT ( 'NONE',  ( 45.44350069997230435, 168.6907664596095344, 34.02200722522286469 ) ) ;
#16064=DIRECTION ( 'NONE',  ( -7.125109674025824596E-05, 0.9999848031710253382, -0.005512562950849464634 ) ) ;
#16120=VERTEX_POINT ( 'NONE', #21409 ) ;
#16201=CIRCLE ( 'NONE', #6989, 4.500000000000006217 ) ;
#16248=LINE ( 'NONE', #7597, #18762 ) ;
#16330=VECTOR ( 'NONE', #7545, 999.9999999999998863 ) ;
#16361=DIRECTION ( 'NONE',  ( -7.125109674025824596E-05, 0.9999848031710253382, -0.005512562950849464634 ) ) ;
#16369=DIRECTION ( 'NONE',  ( -0.01292394549866741384, -0.005513023399720269613, -0.9999012842304692006 ) ) ;
#16374=ORIENTED_EDGE ( 'NONE', *, *, #13140, .T. ) ;
#16395=VERTEX_POINT ( 'NONE', #4851 ) ;
#16447=UNCERTAINTY_MEASURE_WITH_UNIT (LENGTH_MEASURE( 1.000000000000000082E-05 ), #13592, 'distance_accuracy_value', 'NONE');
#16456=ORIENTED_EDGE ( 'NONE', *, *, #11216, .F. ) ;
#16460=APPLICATION_CONTEXT ( 'automotive_design' ) ;
#16470=EDGE_LOOP ( 'NONE', ( #357, #3509, #5302, #993 ) ) ;
#16471=ADVANCED_FACE ( 'NONE', ( #12451, #8637 ), #1998, .F. ) ;
#16518=ADVANCED_FACE ( 'NONE', ( #162, #3924, #5192 ), #3589, .T. ) ;
#16598=CIRCLE ( 'NONE', #16948, 4.500000000000006217 ) ;
#16666=DIRECTION ( 'NONE',  ( -7.125109674118361251E-05, 0.9999848031710253382, -0.005512562950849477644 ) ) ;
#16685=ADVANCED_FACE ( 'NONE', ( #8385 ), #6562, .F. ) ;
#16707=EDGE_LOOP ( 'NONE', ( #8274, #1015, #15055, #10995 ) ) ;
#16760=EDGE_CURVE ( 'NONE', #8927, #6699, #22062, .T. ) ;
#16785=VERTEX_POINT ( 'NONE', #1305 ) ;
#16793=EDGE_LOOP ( 'NONE', ( #21166, #17757, #9442, #15762 ) ) ;
#16802=DIRECTION ( 'NONE',  ( -0.01292394549866741384, -0.005513023399720269613, -0.9999012842304692006 ) ) ;
#16919=CARTESIAN_POINT ( 'NONE',  ( 45.23671757199362986, 168.6025580852140138, 18.02358667753535926 ) ) ;
#16948=AXIS2_PLACEMENT_3D ( 'NONE', #13244, #9676, #716 ) ;
#16983=EDGE_CURVE ( 'NONE', #10445, #8451, #12199, .T. ) ;
#17015=CARTESIAN_POINT ( 'NONE',  ( -44.65237404513518271, 168.6466622724118452, 27.18596972279685531 ) ) ;
#17060=AXIS2_PLACEMENT_3D ( 'NONE', #2189, #4250, #16361 ) ;
#17070=ORIENTED_EDGE ( 'NONE', *, *, #16983, .T. ) ;
#17135=ORIENTED_EDGE ( 'NONE', *, *, #15583, .F. ) ;
#17138=ADVANCED_FACE ( 'NONE', ( #4422, #11114, #2724 ), #18135, .F. ) ;
#17206=ORIENTED_EDGE ( 'NONE', *, *, #8656, .T. ) ;
#17210=FACE_OUTER_BOUND ( 'NONE', #6262, .T. ) ;
#17313=VECTOR ( 'NONE', #21320, 999.9999999999998863 ) ;
#17319=ORIENTED_EDGE ( 'NONE', *, *, #16760, .T. ) ;
#17335=MANIFOLD_SOLID_BREP ( 'Stock-MAS-425-1', #3262 ) ;
#17358=ORIENTED_EDGE ( 'NONE', *, *, #15094, .T. ) ;
#17448=FACE_BOUND ( 'NONE', #22213, .T. ) ;
#17552=ORIENTED_EDGE ( 'NONE', *, *, #7956, .F. ) ;
#17565=VECTOR ( 'NONE', #12484, 999.9999999999998863 ) ;
#17647=( LENGTH_UNIT ( ) NAMED_UNIT ( * ) SI_UNIT ( .MILLI., .METRE. ) );
#17668=CARTESIAN_POINT ( 'NONE',  ( -44.54898248114584192, 168.6907664596095913, 35.18517999664060625 ) ) ;
#17687=CARTESIAN_POINT ( 'NONE',  ( -44.75629999235007972, 176.1024441089967638, 19.14541522682172925 ) ) ;
#17757=ORIENTED_EDGE ( 'NONE', *, *, #10529, .F. ) ;
#17770=AXIS2_PLACEMENT_3D ( 'NONE', #7827, #11381, #13021 ) ;
#17840=DIRECTION ( 'NONE',  ( -0.9999164797902015955, 8.863511990578707937E-16, 0.01292414190464158050 ) ) ;
#17886=DIRECTION ( 'NONE',  ( -0.01292394549866741384, -0.005513023399720269613, -0.9999012842304692006 ) ) ;
#17908=VERTEX_POINT ( 'NONE', #20439 ) ;
#17954=CYLINDRICAL_SURFACE ( 'NONE', #17770, 7.499999999999992006 ) ;
#17967=CIRCLE ( 'NONE', #18674, 4.500000000000006217 ) ;
#18079=AXIS2_PLACEMENT_3D ( 'NONE', #2386, #2488, #896 ) ;
#18135=PLANE ( 'NONE',  #18079 ) ;
#18160=CARTESIAN_POINT ( 'NONE',  ( 45.23671757199362986, 168.6025580852140138, 18.02358667753535926 ) ) ;
#18330=CARTESIAN_POINT ( 'NONE',  ( 45.34042976591830154, 164.1467306581421610, 26.04760348465793385 ) ) ;
#18345=EDGE_CURVE ( 'NONE', #5948, #12252, #22005, .T. ) ;
#18452=CARTESIAN_POINT ( 'NONE',  ( 45.23618318876806654, 176.1024441089967070, 17.98224245540398769 ) ) ;
#18469=EDGE_CURVE ( 'NONE', #16395, #11456, #9603, .T. ) ;
#18549=PRODUCT ( 'Jaw', 'Jaw', '', ( #8359 ) ) ;
#18562=LINE ( 'NONE', #18452, #5241 ) ;
#18618=FACE_OUTER_BOUND ( 'NONE', #8802, .T. ) ;
#18665=FACE_OUTER_BOUND ( 'NONE', #16707, .T. ) ;
#18674=AXIS2_PLACEMENT_3D ( 'NONE', #17015, #2858, #14952 ) ;
#18682=MECHANICAL_DESIGN_GEOMETRIC_PRESENTATION_REPRESENTATION('',(#8763),#5473);
#18701=PRODUCT_DEFINITION ( 'UNKNOWN', '', #13242, #10186 ) ;
#18712=CARTESIAN_POINT ( 'NONE',  ( -44.75523122589896019, 161.1026720614313774, 19.22810367108447238 ) ) ;
#18762=VECTOR ( 'NONE', #5869, 999.9999999999998863 ) ;
#18773=EDGE_LOOP ( 'NONE', ( #6524, #12302 ) ) ;
#18782=ORIENTED_EDGE ( 'NONE', *, *, #1910, .T. ) ;
#18879=EDGE_CURVE ( 'NONE', #13637, #5948, #5024, .T. ) ;
#18895=CARTESIAN_POINT ( 'NONE',  ( 45.23671757199362986, 168.6025580852140138, 18.02358667753535926 ) ) ;
#18906=EDGE_CURVE ( 'NONE', #12945, #7407, #20998, .T. ) ;
#18985=VERTEX_POINT ( 'NONE', #7104 ) ;
#18998=CARTESIAN_POINT ( 'NONE',  ( -44.75576560912451640, 168.6025580852140706, 19.18675944895310082 ) ) ;
#19233=CARTESIAN_POINT ( 'NONE',  ( 45.33957475275741444, 176.1465482961944815, 25.98145272924774218 ) ) ;
#19276=CARTESIAN_POINT ( 'NONE',  ( 67.23320572660466610, 192.1022009597330680, 17.60971032628828681 ) ) ;
#19321=CYLINDRICAL_SURFACE ( 'NONE', #2299, 7.499999999999992006 ) ;
#19391=AXIS2_PLACEMENT_3D ( 'NONE', #20906, #1846, #4939 ) ;
#19467=EDGE_CURVE ( 'NONE', #4369, #17908, #15192, .T. ) ;
#19527=EDGE_CURVE ( 'NONE', #6141, #6699, #18562, .T. ) ;
#19532=AXIS2_PLACEMENT_3D ( 'NONE', #15747, #8696, #6654 ) ;
#19645=EDGE_LOOP ( 'NONE', ( #7027, #5779, #5699, #10944 ) ) ;
#19694=DIRECTION ( 'NONE',  ( -0.01292394549866741384, -0.005513023399720269613, -0.9999012842304692006 ) ) ;
#19733=FACE_OUTER_BOUND ( 'NONE', #6066, .T. ) ;
#19759=ADVANCED_BREP_SHAPE_REPRESENTATION ( '', ( #17335, #6292 ), #1540 ) ;
#19803=CIRCLE ( 'NONE', #15814, 7.499999999999992006 ) ;
#19835=ORIENTED_EDGE ( 'NONE', *, *, #10529, .T. ) ;
#19839=FACE_OUTER_BOUND ( 'NONE', #16470, .T. ) ;
#19850=CARTESIAN_POINT ( 'NONE',  ( 67.23320572660466610, 192.1022009597330680, 17.60971032628828681 ) ) ;
#19947=AXIS2_PLACEMENT_3D ( 'NONE', #1475, #15503, #22454 ) ;
#19953=AXIS2_PLACEMENT_3D ( 'NONE', #5244, #12289, #15511 ) ;
#19960=DIRECTION ( 'NONE',  ( 7.125109674081160920E-05, -0.9999848031710253382, 0.005512562950849312846 ) ) ;
#20249=ADVANCED_FACE ( 'NONE', ( #14962 ), #17954, .F. ) ;
#20297=EDGE_LOOP ( 'NONE', ( #17552, #13996 ) ) ;
#20349=CARTESIAN_POINT ( 'NONE',  ( -66.75560256528235925, 192.1022009597331817, 19.34154534151025118 ) ) ;
#20376=EDGE_CURVE ( 'NONE', #7407, #20796, #14117, .T. ) ;
#20432=EDGE_LOOP ( 'NONE', ( #20475, #10076 ) ) ;
#20439=CARTESIAN_POINT ( 'NONE',  ( -44.65269467507050649, 173.1465938866814724, 27.16116318951803521 ) ) ;
#20475=ORIENTED_EDGE ( 'NONE', *, *, #2688, .F. ) ;
#20491=CYLINDRICAL_SURFACE ( 'NONE', #9682, 4.500000000000006217 ) ;
#20510=DIRECTION ( 'NONE',  ( -7.125109674025824596E-05, 0.9999848031710253382, -0.005512562950849464634 ) ) ;
#20554=VECTOR ( 'NONE', #21646, 1000.000000000000227 ) ;
#20567=EDGE_CURVE ( 'NONE', #18985, #20796, #429, .T. ) ;
#20652=AXIS2_PLACEMENT_3D ( 'NONE', #17668, #3860, #420 ) ;
#20731=CYLINDRICAL_SURFACE ( 'NONE', #15699, 7.499999999999992006 ) ;
#20796=VERTEX_POINT ( 'NONE', #18330 ) ;
#20906=CARTESIAN_POINT ( 'NONE',  ( -44.54898248114584192, 168.6907664596095913, 35.18517999664060625 ) ) ;
#20925=CARTESIAN_POINT ( 'NONE',  ( -66.54547063575685684, 145.1911235850905371, 35.59905634788768225 ) ) ;
#20998=LINE ( 'NONE', #8363, #6355 ) ;
#21095=FACE_OUTER_BOUND ( 'NONE', #18773, .T. ) ;
#21107=PLANE ( 'NONE',  #19953 ) ;
#21166=ORIENTED_EDGE ( 'NONE', *, *, #6824, .F. ) ;
#21194=LINE ( 'NONE', #5448, #17565 ) ;
#21246=AXIS2_PLACEMENT_3D ( 'NONE', #5799, #19694, #10643 ) ;
#21301=EDGE_CURVE ( 'NONE', #2309, #16120, #16248, .T. ) ;
#21314=EDGE_CURVE ( 'NONE', #18985, #12945, #16598, .T. ) ;
#21320=DIRECTION ( 'NONE',  ( -0.01292394549866741557, -0.005513023399720270480, -0.9999012842304693116 ) ) ;
#21385=AXIS2_PLACEMENT_3D ( 'NONE', #10013, #16802, #10234 ) ;
#21409=CARTESIAN_POINT ( 'NONE',  ( -66.54881943730367766, 192.1904093341287307, 35.33996588919776372 ) ) ;
#21485=DIRECTION ( 'NONE',  ( -7.125109674025824596E-05, 0.9999848031710253382, -0.005512562950849464634 ) ) ;
#21509=CARTESIAN_POINT ( 'NONE',  ( 45.23725195521918607, 161.1026720614313206, 18.06493089966673082 ) ) ;
#21515=FACE_OUTER_BOUND ( 'NONE', #21801, .T. ) ;
#21646=DIRECTION ( 'NONE',  ( 0.9999164797902015955, -8.863511990578706951E-16, -0.01292414190464158050 ) ) ;
#21757=VECTOR ( 'NONE', #4509, 1000.000000000000227 ) ;
#21801=EDGE_LOOP ( 'NONE', ( #11145, #11442, #274, #14696 ) ) ;
#21819=ORIENTED_EDGE ( 'NONE', *, *, #6613, .F. ) ;
#22005=LINE ( 'NONE', #4565, #8134 ) ;
#22062=CIRCLE ( 'NONE', #14413, 7.499999999999992006 ) ;
#22103=ORIENTED_EDGE ( 'NONE', *, *, #5841, .T. ) ;
#22163=CARTESIAN_POINT ( 'NONE',  ( -66.75560256528235925, 192.1022009597331817, 19.34154534151025118 ) ) ;
#22213=EDGE_LOOP ( 'NONE', ( #8909, #21819 ) ) ;
#22264=FACE_OUTER_BOUND ( 'NONE', #2742, .T. ) ;
#22281=PRESENTATION_STYLE_ASSIGNMENT (( #10482 ) ) ;
#22454=DIRECTION ( 'NONE',  ( 7.125109674081160920E-05, -0.9999848031710253382, 0.005512562950849312846 ) ) ;
#22481=VERTEX_POINT ( 'NONE', #10832 ) ;
#22607=FILL_AREA_STYLE ('',( #3223 ) ) ;
#22627=ORIENTED_EDGE ( 'NONE', *, *, #3930, .F. ) ;
ENDSEC;
END-ISO-10303-21;
